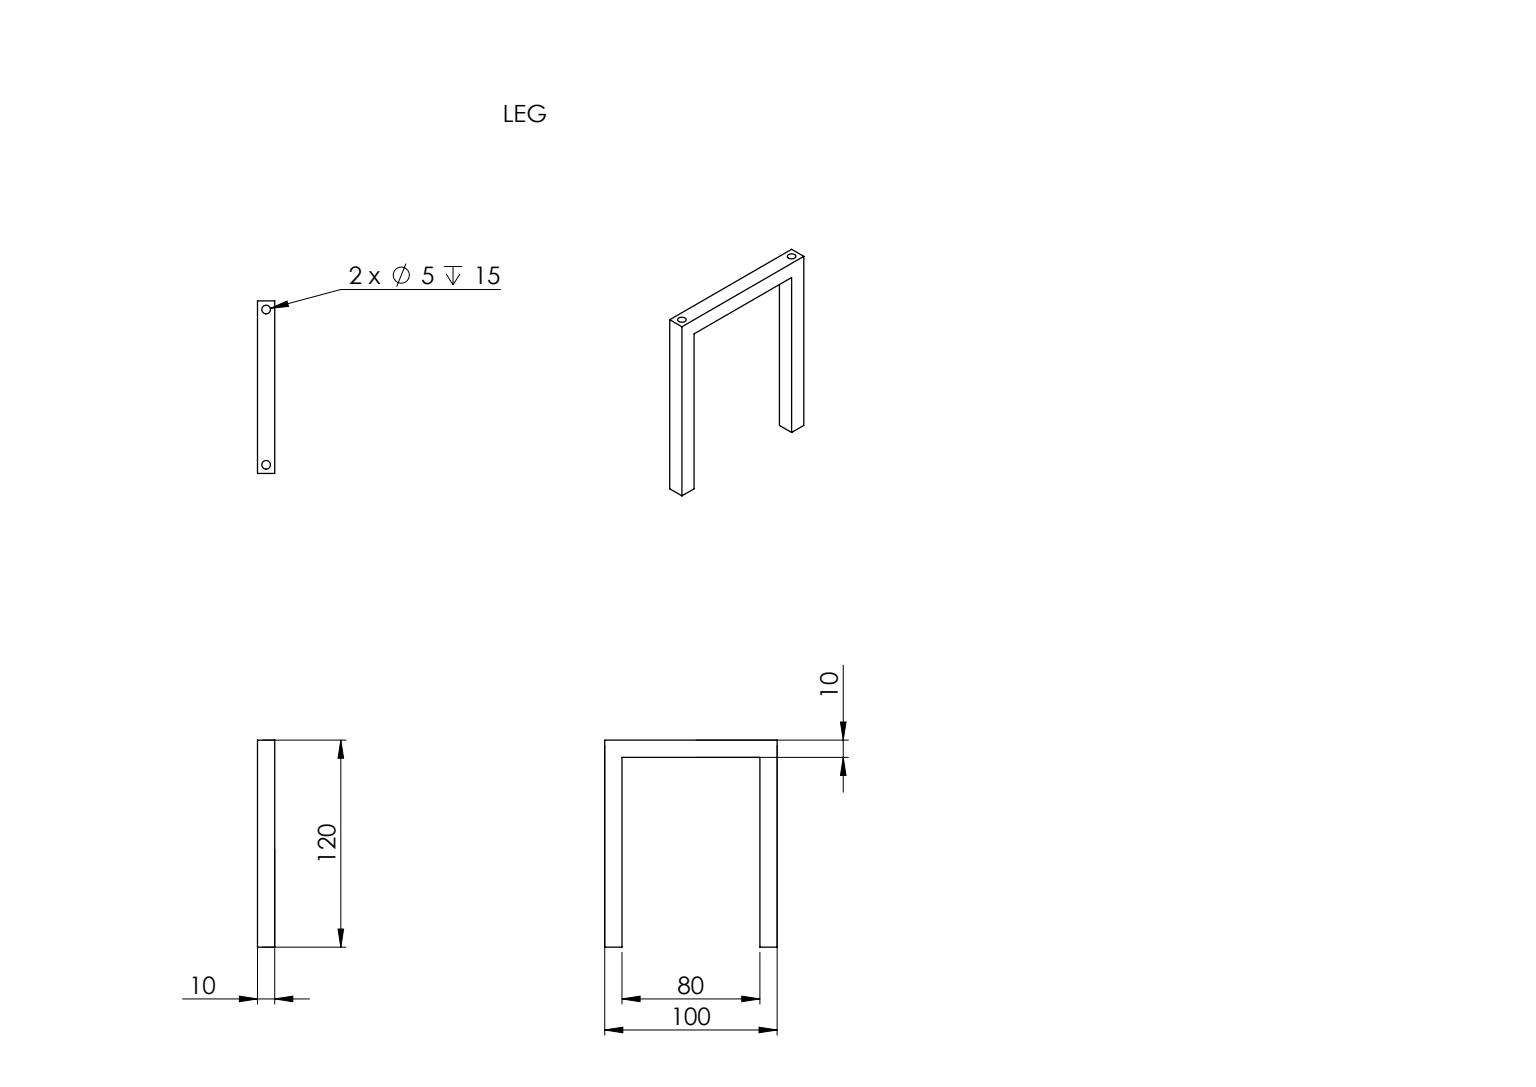
ISO-10303-21;
HEADER;
FILE_DESCRIPTION (('STEP AP214'),
    '1' );
FILE_NAME ('leg.step',
    '2026-10-23T15:04:32',
    ( '' ),
    ( '' ),
    'SwSTEP 2.0',
    'SolidWorks 2026',
    '' );
FILE_SCHEMA (( 'AUTOMOTIVE_DESIGN' ));
ENDSEC;

DATA;
#9=CARTESIAN_POINT ( 'NONE',  ( -145.0000000000000284, -15.00000000000003197, 45.00000000000000000 ) ) ;
#10=EDGE_CURVE ( 'NONE', #1293, #705, #989, .T. ) ;
#12=CIRCLE ( 'NONE', #33, 2.500000000000002220 ) ;
#16=DIRECTION ( 'NONE',  ( -1.000000000000000000, 0.000000000000000000, 0.000000000000000000 ) ) ;
#20=DIRECTION ( 'NONE',  ( 0.000000000000000000, 0.000000000000000000, 1.000000000000000000 ) ) ;
#29=DIRECTION ( 'NONE',  ( -0.000000000000000000, -0.000000000000000000, -1.000000000000000000 ) ) ;
#30=AXIS2_PLACEMENT_3D ( 'NONE', #971, #1660, #79 ) ;
#32=EDGE_LOOP ( 'NONE', ( #1024, #985, #1536, #1885 ) ) ;
#33=AXIS2_PLACEMENT_3D ( 'NONE', #1749, #1441, #229 ) ;
#38=SHAPE_REPRESENTATION ( 'leg', ( #30 ), #544 ) ;
#41=LINE ( 'NONE', #2054, #907 ) ;
#43=CARTESIAN_POINT ( 'NONE',  ( -150.0000000000000000, 0.000000000000000000, 50.00000000000000000 ) ) ;
#45=ORIENTED_EDGE ( 'NONE', *, *, #1333, .T. ) ;
#52=CARTESIAN_POINT ( 'NONE',  ( -145.0000000000000284, -15.00000000000003197, -45.00000000000000000 ) ) ;
#53=EDGE_CURVE ( 'NONE', #738, #333, #1664, .T. ) ;
#56=ORIENTED_EDGE ( 'NONE', *, *, #696, .T. ) ;
#61=CIRCLE ( 'NONE', #2078, 2.500000000000002220 ) ;
#62=DIRECTION ( 'NONE',  ( -0.000000000000000000, 0.000000000000000000, -1.000000000000000000 ) ) ;
#63=LINE ( 'NONE', #106, #788 ) ;
#64=ADVANCED_FACE ( 'NONE', ( #2182 ), #1857, .F. ) ;
#68=ORIENTED_EDGE ( 'NONE', *, *, #53, .F. ) ;
#72=PRODUCT ( 'leg', 'leg', '', ( #943 ) ) ;
#74=ORIENTED_EDGE ( 'NONE', *, *, #1134, .T. ) ;
#79=DIRECTION ( 'NONE',  ( 1.000000000000000000, 0.000000000000000000, 0.000000000000000000 ) ) ;
#81=ORIENTED_EDGE ( 'NONE', *, *, #373, .T. ) ;
#83=FACE_OUTER_BOUND ( 'NONE', #1993, .T. ) ;
#87=FACE_OUTER_BOUND ( 'NONE', #1431, .T. ) ;
#89=DIRECTION ( 'NONE',  ( -0.000000000000000000, 1.000000000000000000, -0.000000000000000000 ) ) ;
#94=VERTEX_POINT ( 'NONE', #1687 ) ;
#96=( LENGTH_UNIT ( ) NAMED_UNIT ( * ) SI_UNIT ( .MILLI., .METRE. ) );
#97=EDGE_LOOP ( 'NONE', ( #511, #45, #1713, #1611, #2168, #1515, #1183, #1829 ) ) ;
#98=AXIS2_PLACEMENT_3D ( 'NONE', #2176, #427, #1287 ) ;
#99=DIRECTION ( 'NONE',  ( 0.000000000000000000, 0.000000000000000000, 1.000000000000000000 ) ) ;
#104=AXIS2_PLACEMENT_3D ( 'NONE', #52, #222, #918 ) ;
#106=CARTESIAN_POINT ( 'NONE',  ( -139.9999999999999716, 2.312964634635743056E-15, -50.00000000000000000 ) ) ;
#108=ORIENTED_EDGE ( 'NONE', *, *, #1169, .T. ) ;
#112=CARTESIAN_POINT ( 'NONE',  ( -139.9999999999999716, 2.312964634635743056E-15, 50.00000000000000000 ) ) ;
#116=ADVANCED_FACE ( 'NONE', ( #1527 ), #1518, .T. ) ;
#124=LINE ( 'NONE', #1842, #1158 ) ;
#125=ORIENTED_EDGE ( 'NONE', *, *, #416, .T. ) ;
#127=LINE ( 'NONE', #2039, #1839 ) ;
#130=DIRECTION ( 'NONE',  ( 0.000000000000000000, -1.000000000000000000, 0.000000000000000000 ) ) ;
#134=DIRECTION ( 'NONE',  ( 2.312964634635742957E-16, -1.000000000000000000, 0.000000000000000000 ) ) ;
#147=DIRECTION ( 'NONE',  ( -1.000000000000000000, 0.000000000000000000, -0.000000000000000000 ) ) ;
#155=AXIS2_PLACEMENT_3D ( 'NONE', #797, #1356, #500 ) ;
#161=UNCERTAINTY_MEASURE_WITH_UNIT (LENGTH_MEASURE( 1.000000000000000082E-05 ), #96, 'distance_accuracy_value', 'NONE');
#173=DIRECTION ( 'NONE',  ( -1.000000000000000000, 0.000000000000000000, 0.000000000000000000 ) ) ;
#175=CLOSED_SHELL ( 'NONE', ( #313, #917, #64, #1213, #1876, #1890, #1705, #1823, #1721, #1503, #2061, #116, #1440, #2153, #1530, #1941, #1489, #1042 ) ) ;
#187=AXIS2_PLACEMENT_3D ( 'NONE', #646, #1683, #147 ) ;
#191=CARTESIAN_POINT ( 'NONE',  ( -145.0000000000000284, -15.00000000000003197, 47.50000000000000000 ) ) ;
#194=CIRCLE ( 'NONE', #1276, 2.500000000000002220 ) ;
#198=DIRECTION ( 'NONE',  ( -0.000000000000000000, 1.000000000000000000, -0.000000000000000000 ) ) ;
#203=AXIS2_PLACEMENT_3D ( 'NONE', #709, #130, #651 ) ;
#208=EDGE_CURVE ( 'NONE', #749, #899, #1717, .T. ) ;
#222=DIRECTION ( 'NONE',  ( -0.000000000000000000, 1.000000000000000000, -0.000000000000000000 ) ) ;
#229=DIRECTION ( 'NONE',  ( 0.000000000000000000, 0.000000000000000000, 1.000000000000000000 ) ) ;
#237=DIRECTION ( 'NONE',  ( -0.000000000000000000, -0.000000000000000000, -1.000000000000000000 ) ) ;
#244=DIRECTION ( 'NONE',  ( -5.046468293750711010E-16, 1.000000000000000000, 0.000000000000000000 ) ) ;
#247=( LENGTH_UNIT ( ) NAMED_UNIT ( * ) SI_UNIT ( .MILLI., .METRE. ) );
#264=SURFACE_STYLE_USAGE ( .BOTH. , #1999 ) ;
#265=ORIENTED_EDGE ( 'NONE', *, *, #1150, .F. ) ;
#268=DIRECTION ( 'NONE',  ( 0.000000000000000000, 0.000000000000000000, -1.000000000000000000 ) ) ;
#269=CARTESIAN_POINT ( 'NONE',  ( -150.0000000000000000, 0.000000000000000000, -50.00000000000000000 ) ) ;
#275=CARTESIAN_POINT ( 'NONE',  ( 0.000000000000000000, 0.000000000000000000, 50.00000000000000000 ) ) ;
#280=ORIENTED_EDGE ( 'NONE', *, *, #988, .T. ) ;
#284=CARTESIAN_POINT ( 'NONE',  ( -145.0000000000000284, -15.00000000000003197, 42.49999999999999289 ) ) ;
#289=DIRECTION ( 'NONE',  ( 0.000000000000000000, 0.000000000000000000, 1.000000000000000000 ) ) ;
#294=ORIENTED_EDGE ( 'NONE', *, *, #359, .T. ) ;
#296=ORIENTED_EDGE ( 'NONE', *, *, #1610, .F. ) ;
#299=DIRECTION ( 'NONE',  ( 0.000000000000000000, 0.5150380749100541555, 0.8571673007021122226 ) ) ;
#309=CARTESIAN_POINT ( 'NONE',  ( -139.9999999999999716, -120.0000000000000142, 40.00000000000000000 ) ) ;
#310=ORIENTED_EDGE ( 'NONE', *, *, #2133, .T. ) ;
#313=ADVANCED_FACE ( 'NONE', ( #1926 ), #1245, .F. ) ;
#324=VERTEX_POINT ( 'NONE', #2098 ) ;
#328=ORIENTED_EDGE ( 'NONE', *, *, #868, .F. ) ;
#333=VERTEX_POINT ( 'NONE', #561 ) ;
#335=CARTESIAN_POINT ( 'NONE',  ( -139.9999999999999716, -120.0000000000000142, 40.00000000000000000 ) ) ;
#340=DIRECTION ( 'NONE',  ( -2.312964634635743450E-16, 1.000000000000000000, 0.000000000000000000 ) ) ;
#347=CARTESIAN_POINT ( 'NONE',  ( -139.9999999999999716, -120.0000000000000142, -40.00000000000000000 ) ) ;
#356=EDGE_CURVE ( 'NONE', #705, #671, #1769, .T. ) ;
#359=EDGE_CURVE ( 'NONE', #738, #1430, #1432, .T. ) ;
#366=CARTESIAN_POINT ( 'NONE',  ( -145.0000000000000284, -16.50215154756893554, 45.00000000000000000 ) ) ;
#372=VECTOR ( 'NONE', #803, 1000.000000000000000 ) ;
#373=EDGE_CURVE ( 'NONE', #1909, #1887, #2134, .T. ) ;
#376=LINE ( 'NONE', #347, #1059 ) ;
#383=DIRECTION ( 'NONE',  ( -0.000000000000000000, 1.000000000000000000, -0.000000000000000000 ) ) ;
#395=AXIS2_PLACEMENT_3D ( 'NONE', #1475, #639, #1634 ) ;
#398=EDGE_LOOP ( 'NONE', ( #310, #2160, #521, #2213 ) ) ;
#403=DIRECTION ( 'NONE',  ( 0.000000000000000000, 0.000000000000000000, 1.000000000000000000 ) ) ;
#404=COLOUR_RGB ( '',0.8941176470588234615, 0.8941176470588234615, 0.8941176470588234615 ) ;
#407=ORIENTED_EDGE ( 'NONE', *, *, #2177, .F. ) ;
#414=LINE ( 'NONE', #1587, #1253 ) ;
#416=EDGE_CURVE ( 'NONE', #94, #899, #2141, .T. ) ;
#421=DIRECTION ( 'NONE',  ( -1.000000000000000000, 0.000000000000000000, 0.000000000000000000 ) ) ;
#422=LINE ( 'NONE', #1104, #878 ) ;
#427=DIRECTION ( 'NONE',  ( 0.000000000000000000, -1.000000000000000000, 0.000000000000000000 ) ) ;
#440=EDGE_LOOP ( 'NONE', ( #687, #1990, #789, #2117 ) ) ;
#445=ORIENTED_EDGE ( 'NONE', *, *, #1312, .T. ) ;
#447=EDGE_LOOP ( 'NONE', ( #2179, #296 ) ) ;
#450=PLANE ( 'NONE',  #98 ) ;
#453=PRODUCT_DEFINITION ( 'UNKNOWN', '', #940, #1003 ) ;
#456=ORIENTED_EDGE ( 'NONE', *, *, #633, .T. ) ;
#459=DIRECTION ( 'NONE',  ( -0.000000000000000000, 1.000000000000000000, -0.000000000000000000 ) ) ;
#466=DIRECTION ( 'NONE',  ( -5.204170427930417339E-16, -1.000000000000000000, 0.000000000000000000 ) ) ;
#472=( NAMED_UNIT ( * ) SI_UNIT ( $, .STERADIAN. ) SOLID_ANGLE_UNIT ( ) );
#474=CARTESIAN_POINT ( 'NONE',  ( -145.0000000000000284, -3.358697307418414604E-14, -47.50000000000000000 ) ) ;
#475=ORIENTED_EDGE ( 'NONE', *, *, #2178, .F. ) ;
#477=EDGE_CURVE ( 'NONE', #333, #2156, #1577, .T. ) ;
#479=DIRECTION ( 'NONE',  ( -0.000000000000000000, 1.000000000000000000, -0.000000000000000000 ) ) ;
#483=ORIENTED_EDGE ( 'NONE', *, *, #1734, .F. ) ;
#485=PLANE ( 'NONE',  #1391 ) ;
#492=CARTESIAN_POINT ( 'NONE',  ( -145.0000000000000284, -3.358697307418414604E-14, 42.49999999999999289 ) ) ;
#496=AXIS2_PLACEMENT_3D ( 'NONE', #1411, #795, #99 ) ;
#500=DIRECTION ( 'NONE',  ( 0.000000000000000000, 0.000000000000000000, 1.000000000000000000 ) ) ;
#502=UNCERTAINTY_MEASURE_WITH_UNIT (LENGTH_MEASURE( 1.000000000000000082E-05 ), #1094, 'distance_accuracy_value', 'NONE');
#506=VECTOR ( 'NONE', #299, 1000.000000000000114 ) ;
#511=ORIENTED_EDGE ( 'NONE', *, *, #1169, .F. ) ;
#516=DIRECTION ( 'NONE',  ( -0.000000000000000000, 1.000000000000000000, -0.000000000000000000 ) ) ;
#521=ORIENTED_EDGE ( 'NONE', *, *, #477, .F. ) ;
#532=LINE ( 'NONE', #1215, #838 ) ;
#533=AXIS2_PLACEMENT_3D ( 'NONE', #1446, #89, #1957 ) ;
#536=AXIS2_PLACEMENT_3D ( 'NONE', #928, #2126, #403 ) ;
#540=CARTESIAN_POINT ( 'NONE',  ( -149.9999999999999716, -120.0000000000000142, -50.00000000000000000 ) ) ;
#541=EDGE_CURVE ( 'NONE', #899, #2107, #1532, .T. ) ;
#544=( GEOMETRIC_REPRESENTATION_CONTEXT ( 3 ) GLOBAL_UNCERTAINTY_ASSIGNED_CONTEXT ( ( #161 ) ) GLOBAL_UNIT_ASSIGNED_CONTEXT ( ( #96, #1865, #2034 ) ) REPRESENTATION_CONTEXT ( 'NONE', 'WORKASPACE' ) );
#545=VECTOR ( 'NONE', #1920, 1000.000000000000000 ) ;
#550=ORIENTED_EDGE ( 'NONE', *, *, #1571, .T. ) ;
#553=PLANE ( 'NONE',  #1005 ) ;
#557=VECTOR ( 'NONE', #16, 1000.000000000000000 ) ;
#561=CARTESIAN_POINT ( 'NONE',  ( -139.9999999999999716, -120.0000000000000142, 50.00000000000000000 ) ) ;
#566=LINE ( 'NONE', #1777, #1649 ) ;
#568=ORIENTED_EDGE ( 'NONE', *, *, #1707, .T. ) ;
#569=AXIS2_PLACEMENT_3D ( 'NONE', #1832, #466, #839 ) ;
#573=CARTESIAN_POINT ( 'NONE',  ( -150.0000000000000284, -9.999999999999994671, -40.00000000000000000 ) ) ;
#579=AXIS2_PLACEMENT_3D ( 'NONE', #9, #516, #20 ) ;
#588=FACE_OUTER_BOUND ( 'NONE', #607, .T. ) ;
#607=EDGE_LOOP ( 'NONE', ( #2150, #1303, #1866, #1115 ) ) ;
#612=ORIENTED_EDGE ( 'NONE', *, *, #1333, .F. ) ;
#615=FACE_BOUND ( 'NONE', #447, .T. ) ;
#623=FACE_OUTER_BOUND ( 'NONE', #1302, .T. ) ;
#625=VERTEX_POINT ( 'NONE', #492 ) ;
#633=EDGE_CURVE ( 'NONE', #860, #2107, #1339, .T. ) ;
#634=ORIENTED_EDGE ( 'NONE', *, *, #1668, .T. ) ;
#639=DIRECTION ( 'NONE',  ( -2.312964634635740985E-16, 1.000000000000000000, 0.000000000000000000 ) ) ;
#642=PRESENTATION_STYLE_ASSIGNMENT (( #264 ) ) ;
#643=VERTEX_POINT ( 'NONE', #2041 ) ;
#644=CONICAL_SURFACE ( 'NONE', #536, 2.500000000000002220, 1.029744258676654534 ) ;
#646=CARTESIAN_POINT ( 'NONE',  ( 0.000000000000000000, 0.000000000000000000, 40.00000000000000000 ) ) ;
#647=EDGE_LOOP ( 'NONE', ( #1594, #634, #74, #1929 ) ) ;
#651=DIRECTION ( 'NONE',  ( 0.000000000000000000, -0.000000000000000000, -1.000000000000000000 ) ) ;
#663=DIRECTION ( 'NONE',  ( -2.312964634635742957E-16, 1.000000000000000000, 0.000000000000000000 ) ) ;
#671=VERTEX_POINT ( 'NONE', #991 ) ;
#675=VECTOR ( 'NONE', #752, 1000.000000000000000 ) ;
#680=VECTOR ( 'NONE', #244, 1000.000000000000000 ) ;
#687=ORIENTED_EDGE ( 'NONE', *, *, #1542, .F. ) ;
#696=EDGE_CURVE ( 'NONE', #324, #1887, #700, .T. ) ;
#698=EDGE_CURVE ( 'NONE', #705, #1125, #1513, .T. ) ;
#700=LINE ( 'NONE', #1557, #545 ) ;
#703=EDGE_CURVE ( 'NONE', #333, #643, #1576, .T. ) ;
#705=VERTEX_POINT ( 'NONE', #191 ) ;
#709=CARTESIAN_POINT ( 'NONE',  ( -139.9999999999999716, -120.0000000000000142, 50.00000000000000000 ) ) ;
#710=ORIENTED_EDGE ( 'NONE', *, *, #1596, .F. ) ;
#719=LINE ( 'NONE', #821, #2072 ) ;
#727=CARTESIAN_POINT ( 'NONE',  ( -145.0000000000000284, -15.00000000000003197, -47.50000000000000000 ) ) ;
#728=ORIENTED_EDGE ( 'NONE', *, *, #10, .F. ) ;
#738=VERTEX_POINT ( 'NONE', #1409 ) ;
#739=CARTESIAN_POINT ( 'NONE',  ( -145.0000000000000284, -3.353798720221824946E-14, -45.00000000000000000 ) ) ;
#741=DIRECTION ( 'NONE',  ( -0.000000000000000000, 1.000000000000000000, -0.000000000000000000 ) ) ;
#742=VECTOR ( 'NONE', #1443, 1000.000000000000000 ) ;
#748=EDGE_CURVE ( 'NONE', #2144, #1284, #1372, .T. ) ;
#749=VERTEX_POINT ( 'NONE', #1910 ) ;
#752=DIRECTION ( 'NONE',  ( -0.000000000000000000, 1.000000000000000000, -0.000000000000000000 ) ) ;
#754=PLANE ( 'NONE',  #1436 ) ;
#758=CARTESIAN_POINT ( 'NONE',  ( -149.9999999999999716, -120.0000000000000142, -40.00000000000000000 ) ) ;
#761=ORIENTED_EDGE ( 'NONE', *, *, #1596, .T. ) ;
#763=DIRECTION ( 'NONE',  ( -0.000000000000000000, -0.000000000000000000, 1.000000000000000000 ) ) ;
#766=ORIENTED_EDGE ( 'NONE', *, *, #903, .F. ) ;
#771=PLANE ( 'NONE',  #1011 ) ;
#774=ORIENTED_EDGE ( 'NONE', *, *, #698, .T. ) ;
#784=DIRECTION ( 'NONE',  ( 0.000000000000000000, 0.000000000000000000, 1.000000000000000000 ) ) ;
#786=FACE_OUTER_BOUND ( 'NONE', #1740, .T. ) ;
#788=VECTOR ( 'NONE', #1825, 1000.000000000000000 ) ;
#789=ORIENTED_EDGE ( 'NONE', *, *, #1610, .T. ) ;
#791=DIRECTION ( 'NONE',  ( -0.000000000000000000, -0.000000000000000000, -1.000000000000000000 ) ) ;
#794=VECTOR ( 'NONE', #237, 1000.000000000000000 ) ;
#795=DIRECTION ( 'NONE',  ( -0.000000000000000000, 1.000000000000000000, -0.000000000000000000 ) ) ;
#797=CARTESIAN_POINT ( 'NONE',  ( -145.0000000000000284, -3.353798720221824946E-14, -45.00000000000000000 ) ) ;
#803=DIRECTION ( 'NONE',  ( 1.000000000000000000, 2.312964634635740985E-16, 0.000000000000000000 ) ) ;
#805=VERTEX_POINT ( 'NONE', #1753 ) ;
#807=CARTESIAN_POINT ( 'NONE',  ( -145.0000000000000284, -3.353798720221824946E-14, 45.00000000000000000 ) ) ;
#821=CARTESIAN_POINT ( 'NONE',  ( -140.0000000000000000, -10.00000000000000000, -40.00000000000000000 ) ) ;
#823=EDGE_CURVE ( 'NONE', #94, #860, #41, .T. ) ;
#829=FACE_OUTER_BOUND ( 'NONE', #1137, .T. ) ;
#832=DIRECTION ( 'NONE',  ( 1.000000000000000000, 2.312964634635743450E-16, -0.000000000000000000 ) ) ;
#834=CARTESIAN_POINT ( 'NONE',  ( -150.0000000000000000, 0.000000000000000000, 50.00000000000000000 ) ) ;
#837=VECTOR ( 'NONE', #173, 1000.000000000000000 ) ;
#838=VECTOR ( 'NONE', #1899, 1000.000000000000114 ) ;
#839=DIRECTION ( 'NONE',  ( 1.000000000000000000, -5.204170427930417339E-16, 0.000000000000000000 ) ) ;
#841=DIRECTION ( 'NONE',  ( 1.000000000000000000, -5.204170427930417339E-16, 0.000000000000000000 ) ) ;
#860=VERTEX_POINT ( 'NONE', #2070 ) ;
#863=DIRECTION ( 'NONE',  ( 0.000000000000000000, 0.000000000000000000, 1.000000000000000000 ) ) ;
#868=EDGE_CURVE ( 'NONE', #749, #94, #532, .T. ) ;
#878=VECTOR ( 'NONE', #1632, 1000.000000000000000 ) ;
#885=AXIS2_PLACEMENT_3D ( 'NONE', #1917, #892, #1378 ) ;
#887=DIRECTION ( 'NONE',  ( 0.000000000000000000, 0.000000000000000000, 1.000000000000000000 ) ) ;
#892=DIRECTION ( 'NONE',  ( -0.000000000000000000, 1.000000000000000000, -0.000000000000000000 ) ) ;
#899=VERTEX_POINT ( 'NONE', #1130 ) ;
#901=CARTESIAN_POINT ( 'NONE',  ( -139.9999999999999716, -120.0000000000000142, 50.00000000000000000 ) ) ;
#903=EDGE_CURVE ( 'NONE', #1057, #2205, #422, .T. ) ;
#906=VECTOR ( 'NONE', #29, 1000.000000000000000 ) ;
#907=VECTOR ( 'NONE', #1714, 1000.000000000000000 ) ;
#911=ORIENTED_EDGE ( 'NONE', *, *, #1571, .F. ) ;
#917=ADVANCED_FACE ( 'NONE', ( #87 ), #1301, .F. ) ;
#918=DIRECTION ( 'NONE',  ( 0.000000000000000000, 0.000000000000000000, 1.000000000000000000 ) ) ;
#923=DIRECTION ( 'NONE',  ( 0.000000000000000000, 0.000000000000000000, 1.000000000000000000 ) ) ;
#925=CYLINDRICAL_SURFACE ( 'NONE', #1837, 2.500000000000002220 ) ;
#928=CARTESIAN_POINT ( 'NONE',  ( -145.0000000000000284, -15.00000000000003197, -45.00000000000000000 ) ) ;
#930=EDGE_LOOP ( 'NONE', ( #1413, #1074 ) ) ;
#932=( GEOMETRIC_REPRESENTATION_CONTEXT ( 3 ) GLOBAL_UNCERTAINTY_ASSIGNED_CONTEXT ( ( #502 ) ) GLOBAL_UNIT_ASSIGNED_CONTEXT ( ( #1094, #1389, #1217 ) ) REPRESENTATION_CONTEXT ( 'NONE', 'WORKASPACE' ) );
#939=LINE ( 'NONE', #758, #680 ) ;
#940=PRODUCT_DEFINITION_FORMATION_WITH_SPECIFIED_SOURCE ( 'ANY', '', #72, .NOT_KNOWN. ) ;
#943=PRODUCT_CONTEXT ( 'NONE', #2073, 'mechanical' ) ;
#947=ORIENTED_EDGE ( 'NONE', *, *, #903, .T. ) ;
#949=CARTESIAN_POINT ( 'NONE',  ( -145.0000000000000284, -3.353798720221824946E-14, 45.00000000000000000 ) ) ;
#951=DIRECTION ( 'NONE',  ( -0.000000000000000000, -0.000000000000000000, -1.000000000000000000 ) ) ;
#958=PLANE ( 'NONE',  #1828 ) ;
#964=APPLICATION_CONTEXT ( 'automotive_design' ) ;
#971=CARTESIAN_POINT ( 'NONE',  ( 0.000000000000000000, 0.000000000000000000, 0.000000000000000000 ) ) ;
#976=AXIS2_PLACEMENT_3D ( 'NONE', #807, #479, #1345 ) ;
#982=PLANE ( 'NONE',  #395 ) ;
#985=ORIENTED_EDGE ( 'NONE', *, *, #1312, .F. ) ;
#988=EDGE_CURVE ( 'NONE', #2205, #1883, #127, .T. ) ;
#989=LINE ( 'NONE', #1174, #506 ) ;
#991=CARTESIAN_POINT ( 'NONE',  ( -145.0000000000000284, -3.358697307418414604E-14, 47.50000000000000000 ) ) ;
#1000=ORIENTED_EDGE ( 'NONE', *, *, #1331, .T. ) ;
#1003=PRODUCT_DEFINITION_CONTEXT ( 'detailed design', #964, 'design' ) ;
#1005=AXIS2_PLACEMENT_3D ( 'NONE', #2215, #1350, #663 ) ;
#1011=AXIS2_PLACEMENT_3D ( 'NONE', #275, #62, #1082 ) ;
#1012=EDGE_LOOP ( 'NONE', ( #1706, #1747, #125 ) ) ;
#1014=DIRECTION ( 'NONE',  ( -0.000000000000000000, -0.000000000000000000, 1.000000000000000000 ) ) ;
#1017=ORIENTED_EDGE ( 'NONE', *, *, #2177, .T. ) ;
#1024=ORIENTED_EDGE ( 'NONE', *, *, #988, .F. ) ;
#1028=ORIENTED_EDGE ( 'NONE', *, *, #2194, .F. ) ;
#1030=DIRECTION ( 'NONE',  ( 1.049727191138618696E-16, 0.5150380749100541555, -0.8571673007021122226 ) ) ;
#1038=ORIENTED_EDGE ( 'NONE', *, *, #2124, .T. ) ;
#1042=ADVANCED_FACE ( 'NONE', ( #829 ), #1175, .F. ) ;
#1043=VECTOR ( 'NONE', #1912, 1000.000000000000000 ) ;
#1056=CARTESIAN_POINT ( 'NONE',  ( -139.9999999999999716, -120.0000000000000142, -50.00000000000000000 ) ) ;
#1057=VERTEX_POINT ( 'NONE', #2006 ) ;
#1058=CARTESIAN_POINT ( 'NONE',  ( -150.0000000000000284, -9.999999999999994671, -40.00000000000000000 ) ) ;
#1059=VECTOR ( 'NONE', #2062, 1000.000000000000000 ) ;
#1064=ORIENTED_EDGE ( 'NONE', *, *, #1150, .T. ) ;
#1068=DIRECTION ( 'NONE',  ( -0.000000000000000000, 0.000000000000000000, -1.000000000000000000 ) ) ;
#1071=CARTESIAN_POINT ( 'NONE',  ( -139.9999999999999716, 2.312964634635743056E-15, 50.00000000000000000 ) ) ;
#1072=LINE ( 'NONE', #1901, #1043 ) ;
#1074=ORIENTED_EDGE ( 'NONE', *, *, #1134, .F. ) ;
#1078=LINE ( 'NONE', #901, #794 ) ;
#1082=DIRECTION ( 'NONE',  ( -1.000000000000000000, 0.000000000000000000, 0.000000000000000000 ) ) ;
#1084=DIRECTION ( 'NONE',  ( -0.000000000000000000, 1.000000000000000000, -0.000000000000000000 ) ) ;
#1094=( LENGTH_UNIT ( ) NAMED_UNIT ( * ) SI_UNIT ( .MILLI., .METRE. ) );
#1095=EDGE_CURVE ( 'NONE', #2156, #1057, #1508, .T. ) ;
#1096=VECTOR ( 'NONE', #763, 1000.000000000000000 ) ;
#1104=CARTESIAN_POINT ( 'NONE',  ( -149.9999999999999716, -120.0000000000000142, 40.00000000000000000 ) ) ;
#1109=FILL_AREA_STYLE ('',( #1814 ) ) ;
#1115=ORIENTED_EDGE ( 'NONE', *, *, #1181, .T. ) ;
#1122=AXIS2_PLACEMENT_3D ( 'NONE', #1784, #2151, #784 ) ;
#1125=VERTEX_POINT ( 'NONE', #1471 ) ;
#1126=CARTESIAN_POINT ( 'NONE',  ( 0.000000000000000000, 0.000000000000000000, -40.00000000000000000 ) ) ;
#1130=CARTESIAN_POINT ( 'NONE',  ( -145.0000000000000284, -15.00000000000003197, -47.50000000000000000 ) ) ;
#1132=FACE_OUTER_BOUND ( 'NONE', #1268, .T. ) ;
#1133=VERTEX_POINT ( 'NONE', #1332 ) ;
#1134=EDGE_CURVE ( 'NONE', #625, #671, #194, .T. ) ;
#1137=EDGE_LOOP ( 'NONE', ( #1401, #1289, #2074, #456 ) ) ;
#1150=EDGE_CURVE ( 'NONE', #1509, #1133, #2069, .T. ) ;
#1152=DIRECTION ( 'NONE',  ( -1.000000000000000000, 0.000000000000000000, 0.000000000000000000 ) ) ;
#1153=CARTESIAN_POINT ( 'NONE',  ( -145.0000000000000284, -3.358697307418414604E-14, -45.00000000000000000 ) ) ;
#1155=SHAPE_DEFINITION_REPRESENTATION ( #1621, #38 ) ;
#1156=( GEOMETRIC_REPRESENTATION_CONTEXT ( 3 ) GLOBAL_UNCERTAINTY_ASSIGNED_CONTEXT ( ( #2211 ) ) GLOBAL_UNIT_ASSIGNED_CONTEXT ( ( #247, #1487, #472 ) ) REPRESENTATION_CONTEXT ( 'NONE', 'WORKASPACE' ) );
#1158=VECTOR ( 'NONE', #791, 1000.000000000000000 ) ;
#1160=DIRECTION ( 'NONE',  ( 1.049727191138618696E-16, 0.5150380749100541555, -0.8571673007021122226 ) ) ;
#1162=ORIENTED_EDGE ( 'NONE', *, *, #208, .T. ) ;
#1169=EDGE_CURVE ( 'NONE', #1509, #1284, #376, .T. ) ;
#1171=CARTESIAN_POINT ( 'NONE',  ( -150.0000000000000284, -9.999999999999994671, -40.00000000000000000 ) ) ;
#1174=CARTESIAN_POINT ( 'NONE',  ( -145.0000000000000284, -15.00000000000003197, 47.50000000000000000 ) ) ;
#1175=CYLINDRICAL_SURFACE ( 'NONE', #155, 2.500000000000002220 ) ;
#1180=FACE_OUTER_BOUND ( 'NONE', #398, .T. ) ;
#1181=EDGE_CURVE ( 'NONE', #671, #625, #1387, .T. ) ;
#1183=ORIENTED_EDGE ( 'NONE', *, *, #1573, .T. ) ;
#1186=DIRECTION ( 'NONE',  ( 2.312964634635742957E-16, -1.000000000000000000, 0.000000000000000000 ) ) ;
#1193=ORIENTED_EDGE ( 'NONE', *, *, #1542, .T. ) ;
#1201=DIRECTION ( 'NONE',  ( 1.000000000000000000, -5.204170427930417339E-16, 0.000000000000000000 ) ) ;
#1213=ADVANCED_FACE ( 'NONE', ( #1574 ), #1852, .F. ) ;
#1215=CARTESIAN_POINT ( 'NONE',  ( -145.0000000000000284, -15.00000000000003197, -42.49999999999999289 ) ) ;
#1217=( NAMED_UNIT ( * ) SI_UNIT ( $, .STERADIAN. ) SOLID_ANGLE_UNIT ( ) );
#1218=ORIENTED_EDGE ( 'NONE', *, *, #2178, .T. ) ;
#1220=CARTESIAN_POINT ( 'NONE',  ( -139.9999999999999716, -120.0000000000000142, -40.00000000000000000 ) ) ;
#1225=VECTOR ( 'NONE', #1671, 1000.000000000000000 ) ;
#1229=LINE ( 'NONE', #43, #2010 ) ;
#1243=ORIENTED_EDGE ( 'NONE', *, *, #2133, .F. ) ;
#1245=CYLINDRICAL_SURFACE ( 'NONE', #2102, 2.500000000000002220 ) ;
#1253=VECTOR ( 'NONE', #1084, 1000.000000000000000 ) ;
#1268=EDGE_LOOP ( 'NONE', ( #407, #911, #1644, #294 ) ) ;
#1276=AXIS2_PLACEMENT_3D ( 'NONE', #1346, #2162, #289 ) ;
#1281=CARTESIAN_POINT ( 'NONE',  ( 0.000000000000000000, 0.000000000000000000, -50.00000000000000000 ) ) ;
#1284=VERTEX_POINT ( 'NONE', #1563 ) ;
#1287=DIRECTION ( 'NONE',  ( 0.000000000000000000, -0.000000000000000000, -1.000000000000000000 ) ) ;
#1289=ORIENTED_EDGE ( 'NONE', *, *, #416, .F. ) ;
#1293=VERTEX_POINT ( 'NONE', #366 ) ;
#1294=CARTESIAN_POINT ( 'NONE',  ( -139.9999999999999716, -120.0000000000000142, -50.00000000000000000 ) ) ;
#1298=FACE_OUTER_BOUND ( 'NONE', #1677, .T. ) ;
#1301=CONICAL_SURFACE ( 'NONE', #1122, 2.500000000000002220, 1.029744258676654534 ) ;
#1302=EDGE_LOOP ( 'NONE', ( #2097, #1843, #947, #280 ) ) ;
#1303=ORIENTED_EDGE ( 'NONE', *, *, #698, .F. ) ;
#1312=EDGE_CURVE ( 'NONE', #2144, #2205, #1965, .T. ) ;
#1324=MECHANICAL_DESIGN_GEOMETRIC_PRESENTATION_REPRESENTATION('',(#1329),#932);
#1329=STYLED_ITEM('',(#2254),#1673);
#1331=EDGE_CURVE ( 'NONE', #1125, #705, #12, .T. ) ;
#1332=CARTESIAN_POINT ( 'NONE',  ( -149.9999999999999716, -120.0000000000000142, -40.00000000000000000 ) ) ;
#1333=EDGE_CURVE ( 'NONE', #1509, #1909, #1078, .T. ) ;
#1336=CARTESIAN_POINT ( 'NONE',  ( -139.9999999999999716, 2.312964634635743056E-15, 50.00000000000000000 ) ) ;
#1339=CIRCLE ( 'NONE', #1406, 2.500000000000002220 ) ;
#1345=DIRECTION ( 'NONE',  ( 0.000000000000000000, 0.000000000000000000, 1.000000000000000000 ) ) ;
#1346=CARTESIAN_POINT ( 'NONE',  ( -145.0000000000000284, -3.358697307418414604E-14, 45.00000000000000000 ) ) ;
#1350=DIRECTION ( 'NONE',  ( 1.000000000000000000, 2.312964634635742957E-16, -0.000000000000000000 ) ) ;
#1356=DIRECTION ( 'NONE',  ( -0.000000000000000000, 1.000000000000000000, -0.000000000000000000 ) ) ;
#1359=DIRECTION ( 'NONE',  ( -0.000000000000000000, 1.000000000000000000, -0.000000000000000000 ) ) ;
#1372=LINE ( 'NONE', #1058, #1692 ) ;
#1378=DIRECTION ( 'NONE',  ( 0.000000000000000000, 0.000000000000000000, 1.000000000000000000 ) ) ;
#1387=CIRCLE ( 'NONE', #1886, 2.500000000000002220 ) ;
#1389=( NAMED_UNIT ( * ) PLANE_ANGLE_UNIT ( ) SI_UNIT ( $, .RADIAN. ) );
#1391=AXIS2_PLACEMENT_3D ( 'NONE', #1336, #832, #340 ) ;
#1401=ORIENTED_EDGE ( 'NONE', *, *, #541, .F. ) ;
#1406=AXIS2_PLACEMENT_3D ( 'NONE', #1153, #1359, #2185 ) ;
#1409=CARTESIAN_POINT ( 'NONE',  ( -139.9999999999999716, 2.312964634635743056E-15, 50.00000000000000000 ) ) ;
#1411=CARTESIAN_POINT ( 'NONE',  ( -145.0000000000000284, -15.00000000000003197, -45.00000000000000000 ) ) ;
#1413=ORIENTED_EDGE ( 'NONE', *, *, #1181, .F. ) ;
#1414=ORIENTED_EDGE ( 'NONE', *, *, #10, .T. ) ;
#1430=VERTEX_POINT ( 'NONE', #1760 ) ;
#1431=EDGE_LOOP ( 'NONE', ( #328, #1162, #1193 ) ) ;
#1432=LINE ( 'NONE', #1071, #1817 ) ;
#1436=AXIS2_PLACEMENT_3D ( 'NONE', #1281, #1068, #421 ) ;
#1440=ADVANCED_FACE ( 'NONE', ( #1806 ), #958, .F. ) ;
#1441=DIRECTION ( 'NONE',  ( -0.000000000000000000, 1.000000000000000000, -0.000000000000000000 ) ) ;
#1443=DIRECTION ( 'NONE',  ( -1.000000000000000000, 0.000000000000000000, 0.000000000000000000 ) ) ;
#1446=CARTESIAN_POINT ( 'NONE',  ( -145.0000000000000284, -15.00000000000003197, 45.00000000000000000 ) ) ;
#1448=VECTOR ( 'NONE', #1152, 1000.000000000000000 ) ;
#1471=CARTESIAN_POINT ( 'NONE',  ( -145.0000000000000284, -15.00000000000003197, 42.49999999999999289 ) ) ;
#1475=CARTESIAN_POINT ( 'NONE',  ( -150.0000000000000000, 0.000000000000000000, 50.00000000000000000 ) ) ;
#1479=EDGE_LOOP ( 'NONE', ( #108, #1803, #483, #265 ) ) ;
#1480=LINE ( 'NONE', #2206, #1225 ) ;
#1487=( NAMED_UNIT ( * ) PLANE_ANGLE_UNIT ( ) SI_UNIT ( $, .RADIAN. ) );
#1489=ADVANCED_FACE ( 'NONE', ( #2114 ), #644, .F. ) ;
#1491=LINE ( 'NONE', #284, #1620 ) ;
#1498=CONICAL_SURFACE ( 'NONE', #533, 2.500000000000002220, 1.029744258676654534 ) ;
#1503=ADVANCED_FACE ( 'NONE', ( #786 ), #771, .F. ) ;
#1508=LINE ( 'NONE', #335, #1448 ) ;
#1509=VERTEX_POINT ( 'NONE', #1947 ) ;
#1513=CIRCLE ( 'NONE', #579, 2.500000000000002220 ) ;
#1515=ORIENTED_EDGE ( 'NONE', *, *, #477, .T. ) ;
#1516=LINE ( 'NONE', #269, #372 ) ;
#1518=PLANE ( 'NONE',  #569 ) ;
#1525=EDGE_LOOP ( 'NONE', ( #710, #1846, #445, #766, #1243, #1652, #550, #56 ) ) ;
#1527=FACE_OUTER_BOUND ( 'NONE', #32, .T. ) ;
#1530=ADVANCED_FACE ( 'NONE', ( #1622 ), #1498, .F. ) ;
#1532=LINE ( 'NONE', #1848, #1875 ) ;
#1536=ORIENTED_EDGE ( 'NONE', *, *, #748, .T. ) ;
#1542=EDGE_CURVE ( 'NONE', #899, #94, #1754, .T. ) ;
#1553=VECTOR ( 'NONE', #134, 1000.000000000000000 ) ;
#1557=CARTESIAN_POINT ( 'NONE',  ( -150.0000000000000000, 0.000000000000000000, -50.00000000000000000 ) ) ;
#1563=CARTESIAN_POINT ( 'NONE',  ( -140.0000000000000000, -10.00000000000000000, -40.00000000000000000 ) ) ;
#1571=EDGE_CURVE ( 'NONE', #805, #324, #1229, .T. ) ;
#1573=EDGE_CURVE ( 'NONE', #2156, #1883, #1072, .T. ) ;
#1574=FACE_OUTER_BOUND ( 'NONE', #1964, .T. ) ;
#1576=LINE ( 'NONE', #2063, #837 ) ;
#1577=LINE ( 'NONE', #2149, #906 ) ;
#1578=DIRECTION ( 'NONE',  ( -0.000000000000000000, -0.000000000000000000, -1.000000000000000000 ) ) ;
#1587=CARTESIAN_POINT ( 'NONE',  ( -145.0000000000000284, -3.353798720221824946E-14, 42.49999999999999289 ) ) ;
#1594=ORIENTED_EDGE ( 'NONE', *, *, #1331, .F. ) ;
#1596=EDGE_CURVE ( 'NONE', #1133, #1887, #566, .T. ) ;
#1602=CARTESIAN_POINT ( 'NONE',  ( -145.0000000000000284, -3.353798720221824946E-14, 47.50000000000000000 ) ) ;
#1610=EDGE_CURVE ( 'NONE', #2107, #860, #61, .T. ) ;
#1611=ORIENTED_EDGE ( 'NONE', *, *, #359, .F. ) ;
#1620=VECTOR ( 'NONE', #1160, 1000.000000000000114 ) ;
#1621=PRODUCT_DEFINITION_SHAPE ( 'NONE', 'NONE',  #453 ) ;
#1622=FACE_OUTER_BOUND ( 'NONE', #2143, .T. ) ;
#1632=DIRECTION ( 'NONE',  ( -5.046468293750711010E-16, 1.000000000000000000, 0.000000000000000000 ) ) ;
#1634=DIRECTION ( 'NONE',  ( -1.000000000000000000, -2.312964634635740985E-16, 0.000000000000000000 ) ) ;
#1639=DIRECTION ( 'NONE',  ( -1.000000000000000000, 0.000000000000000000, -0.000000000000000000 ) ) ;
#1644=ORIENTED_EDGE ( 'NONE', *, *, #2194, .T. ) ;
#1648=VECTOR ( 'NONE', #1186, 1000.000000000000000 ) ;
#1649=VECTOR ( 'NONE', #1756, 1000.000000000000000 ) ;
#1652=ORIENTED_EDGE ( 'NONE', *, *, #2124, .F. ) ;
#1657=MECHANICAL_DESIGN_GEOMETRIC_PRESENTATION_REPRESENTATION('',(#2197),#1156);
#1660=DIRECTION ( 'NONE',  ( 0.000000000000000000, 0.000000000000000000, 1.000000000000000000 ) ) ;
#1664=LINE ( 'NONE', #112, #1648 ) ;
#1667=FACE_OUTER_BOUND ( 'NONE', #97, .T. ) ;
#1668=EDGE_CURVE ( 'NONE', #1125, #625, #414, .T. ) ;
#1671=DIRECTION ( 'NONE',  ( 1.000000000000000000, 2.312964634635740985E-16, 0.000000000000000000 ) ) ;
#1673=MANIFOLD_SOLID_BREP ( 'Tap Drill for M5 Tap2', #175 ) ;
#1677=EDGE_LOOP ( 'NONE', ( #1064, #761, #1695, #612 ) ) ;
#1683=DIRECTION ( 'NONE',  ( 0.000000000000000000, 0.000000000000000000, -1.000000000000000000 ) ) ;
#1687=CARTESIAN_POINT ( 'NONE',  ( -145.0000000000000284, -15.00000000000003197, -42.49999999999999289 ) ) ;
#1692=VECTOR ( 'NONE', #1201, 1000.000000000000000 ) ;
#1695=ORIENTED_EDGE ( 'NONE', *, *, #373, .F. ) ;
#1702=CARTESIAN_POINT ( 'NONE',  ( -139.9999999999999716, -9.999999999999994671, 40.00000000000000000 ) ) ;
#1705=ADVANCED_FACE ( 'NONE', ( #1298 ), #450, .T. ) ;
#1706=ORIENTED_EDGE ( 'NONE', *, *, #208, .F. ) ;
#1707=EDGE_CURVE ( 'NONE', #1430, #1909, #63, .T. ) ;
#1713=ORIENTED_EDGE ( 'NONE', *, *, #1707, .F. ) ;
#1714=DIRECTION ( 'NONE',  ( -0.000000000000000000, 1.000000000000000000, -0.000000000000000000 ) ) ;
#1717=LINE ( 'NONE', #727, #2002 ) ;
#1721=ADVANCED_FACE ( 'NONE', ( #615, #2140, #1132 ), #982, .T. ) ;
#1733=ADVANCED_BREP_SHAPE_REPRESENTATION ( '', ( #1673, #30 ), #544 ) ;
#1734=EDGE_CURVE ( 'NONE', #1133, #2144, #939, .T. ) ;
#1740=EDGE_LOOP ( 'NONE', ( #1038, #1969, #68, #1028 ) ) ;
#1747=ORIENTED_EDGE ( 'NONE', *, *, #868, .T. ) ;
#1749=CARTESIAN_POINT ( 'NONE',  ( -145.0000000000000284, -15.00000000000003197, 45.00000000000000000 ) ) ;
#1753=CARTESIAN_POINT ( 'NONE',  ( -150.0000000000000000, 0.000000000000000000, 50.00000000000000000 ) ) ;
#1754=CIRCLE ( 'NONE', #104, 2.500000000000002220 ) ;
#1756=DIRECTION ( 'NONE',  ( -0.000000000000000000, -0.000000000000000000, -1.000000000000000000 ) ) ;
#1760=CARTESIAN_POINT ( 'NONE',  ( -139.9999999999999716, 2.312964634635743056E-15, -50.00000000000000000 ) ) ;
#1769=LINE ( 'NONE', #1602, #675 ) ;
#1777=CARTESIAN_POINT ( 'NONE',  ( -149.9999999999999716, -120.0000000000000142, 50.00000000000000000 ) ) ;
#1784=CARTESIAN_POINT ( 'NONE',  ( -145.0000000000000284, -15.00000000000003197, -45.00000000000000000 ) ) ;
#1802=EDGE_CURVE ( 'NONE', #1284, #1883, #719, .T. ) ;
#1803=ORIENTED_EDGE ( 'NONE', *, *, #748, .F. ) ;
#1806=FACE_OUTER_BOUND ( 'NONE', #1479, .T. ) ;
#1814=FILL_AREA_STYLE_COLOUR ( '', #404 ) ;
#1817=VECTOR ( 'NONE', #951, 1000.000000000000000 ) ;
#1818=PLANE ( 'NONE',  #187 ) ;
#1823=ADVANCED_FACE ( 'NONE', ( #1667 ), #485, .T. ) ;
#1825=DIRECTION ( 'NONE',  ( 2.312964634635742957E-16, -1.000000000000000000, 0.000000000000000000 ) ) ;
#1828=AXIS2_PLACEMENT_3D ( 'NONE', #1126, #268, #1639 ) ;
#1829=ORIENTED_EDGE ( 'NONE', *, *, #1802, .F. ) ;
#1832=CARTESIAN_POINT ( 'NONE',  ( -150.0000000000000284, -9.999999999999994671, -40.00000000000000000 ) ) ;
#1837=AXIS2_PLACEMENT_3D ( 'NONE', #949, #741, #2110 ) ;
#1839=VECTOR ( 'NONE', #841, 1000.000000000000000 ) ;
#1840=SURFACE_STYLE_FILL_AREA ( #1109 ) ;
#1842=CARTESIAN_POINT ( 'NONE',  ( -149.9999999999999716, -120.0000000000000142, 50.00000000000000000 ) ) ;
#1843=ORIENTED_EDGE ( 'NONE', *, *, #1095, .T. ) ;
#1846=ORIENTED_EDGE ( 'NONE', *, *, #1734, .T. ) ;
#1848=CARTESIAN_POINT ( 'NONE',  ( -145.0000000000000284, -3.353798720221824946E-14, -47.50000000000000000 ) ) ;
#1852=CONICAL_SURFACE ( 'NONE', #885, 2.500000000000002220, 1.029744258676654534 ) ;
#1853=ORIENTED_EDGE ( 'NONE', *, *, #696, .F. ) ;
#1857=CYLINDRICAL_SURFACE ( 'NONE', #976, 2.500000000000002220 ) ;
#1865=( NAMED_UNIT ( * ) PLANE_ANGLE_UNIT ( ) SI_UNIT ( $, .RADIAN. ) );
#1866=ORIENTED_EDGE ( 'NONE', *, *, #356, .T. ) ;
#1875=VECTOR ( 'NONE', #459, 1000.000000000000000 ) ;
#1876=ADVANCED_FACE ( 'NONE', ( #1180 ), #2201, .T. ) ;
#1883=VERTEX_POINT ( 'NONE', #1702 ) ;
#1885=ORIENTED_EDGE ( 'NONE', *, *, #1802, .T. ) ;
#1886=AXIS2_PLACEMENT_3D ( 'NONE', #2221, #198, #863 ) ;
#1887=VERTEX_POINT ( 'NONE', #540 ) ;
#1890=ADVANCED_FACE ( 'NONE', ( #2091 ), #553, .F. ) ;
#1899=DIRECTION ( 'NONE',  ( 0.000000000000000000, 0.5150380749100541555, 0.8571673007021122226 ) ) ;
#1901=CARTESIAN_POINT ( 'NONE',  ( -139.9999999999999716, -120.0000000000000142, 40.00000000000000000 ) ) ;
#1909=VERTEX_POINT ( 'NONE', #1056 ) ;
#1910=CARTESIAN_POINT ( 'NONE',  ( -145.0000000000000284, -16.50215154756893554, -45.00000000000000000 ) ) ;
#1912=DIRECTION ( 'NONE',  ( -5.046468293750711010E-16, 1.000000000000000000, 0.000000000000000000 ) ) ;
#1917=CARTESIAN_POINT ( 'NONE',  ( -145.0000000000000284, -15.00000000000003197, 45.00000000000000000 ) ) ;
#1920=DIRECTION ( 'NONE',  ( 2.312964634635742957E-16, -1.000000000000000000, 0.000000000000000000 ) ) ;
#1926=FACE_OUTER_BOUND ( 'NONE', #440, .T. ) ;
#1929=ORIENTED_EDGE ( 'NONE', *, *, #356, .F. ) ;
#1941=ADVANCED_FACE ( 'NONE', ( #588 ), #925, .F. ) ;
#1947=CARTESIAN_POINT ( 'NONE',  ( -139.9999999999999716, -120.0000000000000142, -40.00000000000000000 ) ) ;
#1957=DIRECTION ( 'NONE',  ( 0.000000000000000000, 0.000000000000000000, 1.000000000000000000 ) ) ;
#1964=EDGE_LOOP ( 'NONE', ( #728, #1218, #1000 ) ) ;
#1965=LINE ( 'NONE', #573, #1096 ) ;
#1969=ORIENTED_EDGE ( 'NONE', *, *, #703, .F. ) ;
#1990=ORIENTED_EDGE ( 'NONE', *, *, #541, .T. ) ;
#1993=EDGE_LOOP ( 'NONE', ( #1853, #1017, #568, #81 ) ) ;
#1999=SURFACE_SIDE_STYLE ('',( #1840 ) ) ;
#2002=VECTOR ( 'NONE', #1030, 1000.000000000000114 ) ;
#2003=CARTESIAN_POINT ( 'NONE',  ( -150.0000000000000284, -9.999999999999994671, 40.00000000000000000 ) ) ;
#2006=CARTESIAN_POINT ( 'NONE',  ( -149.9999999999999716, -120.0000000000000142, 40.00000000000000000 ) ) ;
#2009=SHAPE_REPRESENTATION_RELATIONSHIP ( 'NONE' , 'NONE' ,  #38, #1733 ) ;
#2010=VECTOR ( 'NONE', #1578, 1000.000000000000000 ) ;
#2024=LINE ( 'NONE', #834, #1553 ) ;
#2034=( NAMED_UNIT ( * ) SI_UNIT ( $, .STERADIAN. ) SOLID_ANGLE_UNIT ( ) );
#2039=CARTESIAN_POINT ( 'NONE',  ( -150.0000000000000284, -9.999999999999994671, 40.00000000000000000 ) ) ;
#2041=CARTESIAN_POINT ( 'NONE',  ( -149.9999999999999716, -120.0000000000000142, 50.00000000000000000 ) ) ;
#2054=CARTESIAN_POINT ( 'NONE',  ( -145.0000000000000284, -3.353798720221824946E-14, -42.49999999999999289 ) ) ;
#2061=ADVANCED_FACE ( 'NONE', ( #83 ), #754, .T. ) ;
#2062=DIRECTION ( 'NONE',  ( -5.046468293750711010E-16, 1.000000000000000000, 0.000000000000000000 ) ) ;
#2063=CARTESIAN_POINT ( 'NONE',  ( -139.9999999999999716, -120.0000000000000142, 50.00000000000000000 ) ) ;
#2069=LINE ( 'NONE', #1220, #557 ) ;
#2070=CARTESIAN_POINT ( 'NONE',  ( -145.0000000000000284, -3.358697307418414604E-14, -42.49999999999999289 ) ) ;
#2072=VECTOR ( 'NONE', #1014, 1000.000000000000000 ) ;
#2073=APPLICATION_CONTEXT ( 'automotive_design' ) ;
#2074=ORIENTED_EDGE ( 'NONE', *, *, #823, .T. ) ;
#2078=AXIS2_PLACEMENT_3D ( 'NONE', #2082, #383, #887 ) ;
#2082=CARTESIAN_POINT ( 'NONE',  ( -145.0000000000000284, -3.358697307418414604E-14, -45.00000000000000000 ) ) ;
#2091=FACE_OUTER_BOUND ( 'NONE', #1525, .T. ) ;
#2097=ORIENTED_EDGE ( 'NONE', *, *, #1573, .F. ) ;
#2098=CARTESIAN_POINT ( 'NONE',  ( -150.0000000000000000, 0.000000000000000000, -50.00000000000000000 ) ) ;
#2102=AXIS2_PLACEMENT_3D ( 'NONE', #739, #2118, #923 ) ;
#2107=VERTEX_POINT ( 'NONE', #474 ) ;
#2110=DIRECTION ( 'NONE',  ( 0.000000000000000000, 0.000000000000000000, 1.000000000000000000 ) ) ;
#2114=FACE_OUTER_BOUND ( 'NONE', #1012, .T. ) ;
#2117=ORIENTED_EDGE ( 'NONE', *, *, #823, .F. ) ;
#2118=DIRECTION ( 'NONE',  ( -0.000000000000000000, 1.000000000000000000, -0.000000000000000000 ) ) ;
#2124=EDGE_CURVE ( 'NONE', #805, #643, #2024, .T. ) ;
#2126=DIRECTION ( 'NONE',  ( -0.000000000000000000, 1.000000000000000000, -0.000000000000000000 ) ) ;
#2133=EDGE_CURVE ( 'NONE', #643, #1057, #124, .T. ) ;
#2134=LINE ( 'NONE', #1294, #742 ) ;
#2140=FACE_BOUND ( 'NONE', #930, .T. ) ;
#2141=CIRCLE ( 'NONE', #496, 2.500000000000002220 ) ;
#2143=EDGE_LOOP ( 'NONE', ( #475, #1414, #774 ) ) ;
#2144=VERTEX_POINT ( 'NONE', #1171 ) ;
#2149=CARTESIAN_POINT ( 'NONE',  ( -139.9999999999999716, -120.0000000000000142, 50.00000000000000000 ) ) ;
#2150=ORIENTED_EDGE ( 'NONE', *, *, #1668, .F. ) ;
#2151=DIRECTION ( 'NONE',  ( -0.000000000000000000, 1.000000000000000000, -0.000000000000000000 ) ) ;
#2153=ADVANCED_FACE ( 'NONE', ( #623 ), #1818, .T. ) ;
#2156=VERTEX_POINT ( 'NONE', #309 ) ;
#2160=ORIENTED_EDGE ( 'NONE', *, *, #1095, .F. ) ;
#2162=DIRECTION ( 'NONE',  ( -0.000000000000000000, 1.000000000000000000, -0.000000000000000000 ) ) ;
#2168=ORIENTED_EDGE ( 'NONE', *, *, #53, .T. ) ;
#2176=CARTESIAN_POINT ( 'NONE',  ( -139.9999999999999716, -120.0000000000000142, 50.00000000000000000 ) ) ;
#2177=EDGE_CURVE ( 'NONE', #324, #1430, #1516, .T. ) ;
#2178=EDGE_CURVE ( 'NONE', #1293, #1125, #1491, .T. ) ;
#2179=ORIENTED_EDGE ( 'NONE', *, *, #633, .F. ) ;
#2182=FACE_OUTER_BOUND ( 'NONE', #647, .T. ) ;
#2185=DIRECTION ( 'NONE',  ( 0.000000000000000000, 0.000000000000000000, 1.000000000000000000 ) ) ;
#2194=EDGE_CURVE ( 'NONE', #805, #738, #1480, .T. ) ;
#2197=STYLED_ITEM ( 'NONE', ( #642 ), #1733 ) ;
#2201=PLANE ( 'NONE',  #203 ) ;
#2205=VERTEX_POINT ( 'NONE', #2003 ) ;
#2206=CARTESIAN_POINT ( 'NONE',  ( -150.0000000000000000, 0.000000000000000000, 50.00000000000000000 ) ) ;
#2211=UNCERTAINTY_MEASURE_WITH_UNIT (LENGTH_MEASURE( 1.000000000000000082E-05 ), #247, 'distance_accuracy_value', 'NONE');
#2213=ORIENTED_EDGE ( 'NONE', *, *, #703, .T. ) ;
#2215=CARTESIAN_POINT ( 'NONE',  ( -150.0000000000000000, 0.000000000000000000, 50.00000000000000000 ) ) ;
#2221=CARTESIAN_POINT ( 'NONE',  ( -145.0000000000000284, -3.358697307418414604E-14, 45.00000000000000000 ) ) ;
#2248=COLOUR_RGB('Sky Blue',0.24,0.69,0.87);
#2249=FILL_AREA_STYLE_COLOUR('',#2248);
#2250=FILL_AREA_STYLE('',(#2249));
#2251=SURFACE_STYLE_FILL_AREA(#2250);
#2252=SURFACE_SIDE_STYLE('',(#2251));
#2253=SURFACE_STYLE_USAGE(.BOTH.,#2252);
#2254=PRESENTATION_STYLE_ASSIGNMENT((#2253));
ENDSEC;
END-ISO-10303-21;
